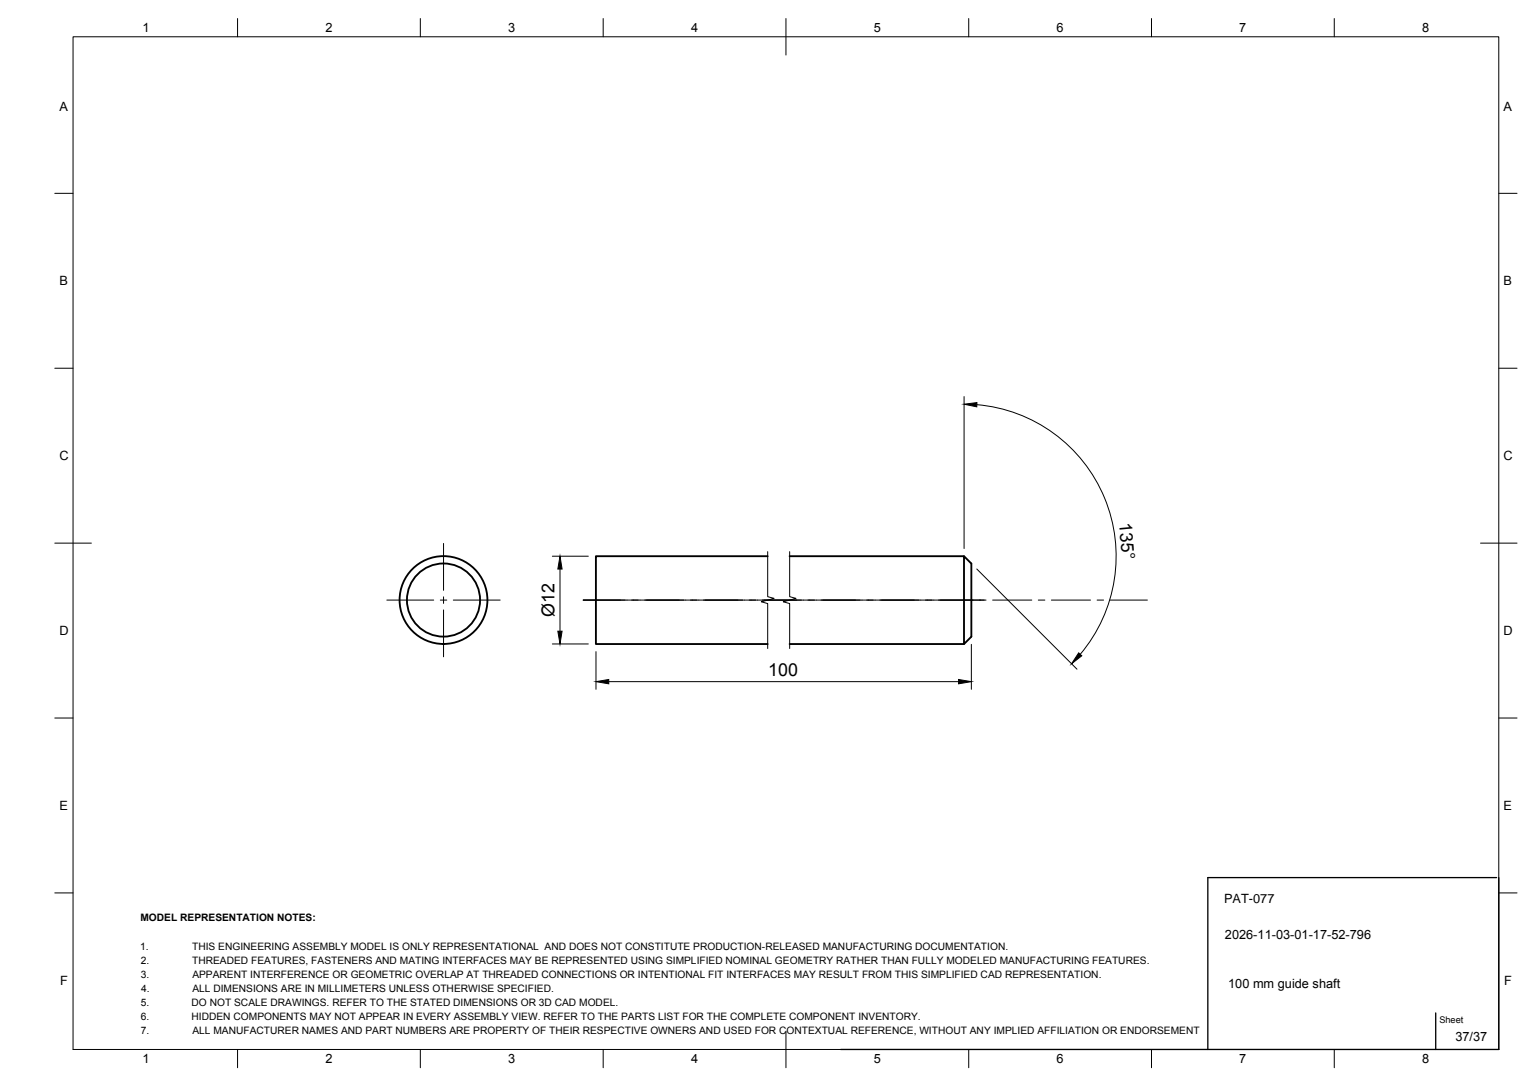
ISO-10303-21;
HEADER;
/* Generated by software containing ST-Developer
 * from STEP Tools, Inc. (www.steptools.com) 
 */

FILE_DESCRIPTION(
/* description */ ('Pallet stop with pneumatic fitting'),
/* implementation_level */ '2;1');

FILE_NAME(
/* name */ '100 mm guide shaft.step',
/* time_stamp */ '2026-10-27T10:51:41-07:00',
/* author */ (''),
/* organization */ (''),
/* preprocessor_version */ 'ST-DEVELOPER v20.2',
/* originating_system */ 'Autodesk Translation Framework v15.17.0.0',
/* authorisation */ '');

FILE_SCHEMA (('AUTOMOTIVE_DESIGN { 1 0 10303 214 3 1 1 }'));
ENDSEC;

DATA;
#10=MECHANICAL_DESIGN_GEOMETRIC_PRESENTATION_REPRESENTATION('',(#386),#10265);
#32=CONICAL_SURFACE('',#5987,0.55,0.785398163397448);
#322=SHAPE_REPRESENTATION_RELATIONSHIP('SRR','None',#10438,#354);
#354=ADVANCED_BREP_SHAPE_REPRESENTATION('',(#417),#10262);
#386=STYLED_ITEM('',(#10655),#417);
#417=MANIFOLD_SOLID_BREP('Body1',#5075);
#714=PLANE('',#5985);
#715=PLANE('',#5991);
#1018=FACE_OUTER_BOUND('',#1456,.T.);
#1019=FACE_OUTER_BOUND('',#1457,.T.);
#1020=FACE_OUTER_BOUND('',#1458,.T.);
#1021=FACE_OUTER_BOUND('',#1459,.T.);
#1456=EDGE_LOOP('',(#4502));
#1457=EDGE_LOOP('',(#4503,#4504,#4505,#4506));
#1458=EDGE_LOOP('',(#4507,#4508,#4509,#4510));
#1459=EDGE_LOOP('',(#4511));
#1779=LINE('',#10009,#2114);
#1780=LINE('',#10012,#2115);
#2114=VECTOR('',#7492,0.55);
#2115=VECTOR('',#7497,0.6);
#2393=CIRCLE('',#5986,0.6);
#2394=CIRCLE('',#5988,0.6);
#2395=CIRCLE('',#5989,0.5);
#2766=VERTEX_POINT('',#10003);
#2767=VERTEX_POINT('',#10006);
#2768=VERTEX_POINT('',#10008);
#3350=EDGE_CURVE('',#2766,#2766,#2393,.T.);
#3351=EDGE_CURVE('',#2767,#2767,#2394,.T.);
#3352=EDGE_CURVE('',#2767,#2768,#1779,.T.);
#3353=EDGE_CURVE('',#2768,#2768,#2395,.T.);
#3354=EDGE_CURVE('',#2766,#2767,#1780,.T.);
#4502=ORIENTED_EDGE('',*,*,#3350,.F.);
#4503=ORIENTED_EDGE('',*,*,#3351,.T.);
#4504=ORIENTED_EDGE('',*,*,#3352,.T.);
#4505=ORIENTED_EDGE('',*,*,#3353,.T.);
#4506=ORIENTED_EDGE('',*,*,#3352,.F.);
#4507=ORIENTED_EDGE('',*,*,#3350,.T.);
#4508=ORIENTED_EDGE('',*,*,#3354,.T.);
#4509=ORIENTED_EDGE('',*,*,#3351,.F.);
#4510=ORIENTED_EDGE('',*,*,#3354,.F.);
#4511=ORIENTED_EDGE('',*,*,#3353,.F.);
#4727=CYLINDRICAL_SURFACE('',#5990,0.6);
#5013=ADVANCED_FACE('',(#1018),#714,.T.);
#5014=ADVANCED_FACE('',(#1019),#32,.T.);
#5015=ADVANCED_FACE('',(#1020),#4727,.T.);
#5016=ADVANCED_FACE('',(#1021),#715,.F.);
#5075=CLOSED_SHELL('',(#5013,#5014,#5015,#5016));
#5984=AXIS2_PLACEMENT_3D('',#10001,#7482,#7483);
#5985=AXIS2_PLACEMENT_3D('',#10002,#7484,#7485);
#5986=AXIS2_PLACEMENT_3D('',#10004,#7486,#7487);
#5987=AXIS2_PLACEMENT_3D('',#10005,#7488,#7489);
#5988=AXIS2_PLACEMENT_3D('',#10007,#7490,#7491);
#5989=AXIS2_PLACEMENT_3D('',#10010,#7493,#7494);
#5990=AXIS2_PLACEMENT_3D('',#10011,#7495,#7496);
#5991=AXIS2_PLACEMENT_3D('',#10013,#7498,#7499);
#7482=DIRECTION('axis',(0.,0.,1.));
#7483=DIRECTION('refdir',(1.,0.,0.));
#7484=DIRECTION('center_axis',(1.,0.,0.));
#7485=DIRECTION('ref_axis',(0.,0.,-1.));
#7486=DIRECTION('center_axis',(-1.,0.,0.));
#7487=DIRECTION('ref_axis',(0.,0.,-1.));
#7488=DIRECTION('center_axis',(1.,0.,0.));
#7489=DIRECTION('ref_axis',(0.,0.,-1.));
#7490=DIRECTION('center_axis',(-1.,0.,0.));
#7491=DIRECTION('ref_axis',(0.,0.,-1.));
#7492=DIRECTION('',(-0.707106781186548,8.65956056235493E-17,-0.707106781186547));
#7493=DIRECTION('center_axis',(1.,0.,0.));
#7494=DIRECTION('ref_axis',(0.,0.,-1.));
#7495=DIRECTION('center_axis',(1.,0.,0.));
#7496=DIRECTION('ref_axis',(0.,0.,-1.));
#7497=DIRECTION('',(-1.,0.,0.));
#7498=DIRECTION('center_axis',(1.,0.,0.));
#7499=DIRECTION('ref_axis',(0.,0.,-1.));
#10001=CARTESIAN_POINT('',(0.,0.,0.));
#10002=CARTESIAN_POINT('Origin',(10.,0.,0.));
#10003=CARTESIAN_POINT('',(10.,7.34788079488412E-17,0.6));
#10004=CARTESIAN_POINT('Origin',(10.,0.,0.));
#10005=CARTESIAN_POINT('Origin',(0.05,0.,0.));
#10006=CARTESIAN_POINT('',(0.1,7.34788079488412E-17,0.6));
#10007=CARTESIAN_POINT('Origin',(0.1,0.,0.));
#10008=CARTESIAN_POINT('',(0.,-6.12323399573677E-17,0.5));
#10009=CARTESIAN_POINT('',(0.05,-6.73555739531044E-17,0.55));
#10010=CARTESIAN_POINT('Origin',(0.,0.,0.));
#10011=CARTESIAN_POINT('Origin',(0.,0.,0.));
#10012=CARTESIAN_POINT('',(0.,-7.34788079488412E-17,0.6));
#10013=CARTESIAN_POINT('Origin',(0.,0.,0.));
#10224=UNCERTAINTY_MEASURE_WITH_UNIT(LENGTH_MEASURE(0.001),#10266,
'DISTANCE_ACCURACY_VALUE',
'Maximum model space distance between geometric entities at asserted c
onnectivities');
#10227=UNCERTAINTY_MEASURE_WITH_UNIT(LENGTH_MEASURE(0.001),#10266,
'DISTANCE_ACCURACY_VALUE',
'Maximum model space distance between geometric entities at asserted c
onnectivities');
#10262=(
GEOMETRIC_REPRESENTATION_CONTEXT(3)
GLOBAL_UNCERTAINTY_ASSIGNED_CONTEXT((#10224))
GLOBAL_UNIT_ASSIGNED_CONTEXT((#10266,#10268,#10269))
REPRESENTATION_CONTEXT('','3D')
);
#10265=(
GEOMETRIC_REPRESENTATION_CONTEXT(3)
GLOBAL_UNCERTAINTY_ASSIGNED_CONTEXT((#10227))
GLOBAL_UNIT_ASSIGNED_CONTEXT((#10266,#10268,#10269))
REPRESENTATION_CONTEXT('','3D')
);
#10266=(
LENGTH_UNIT()
NAMED_UNIT(*)
SI_UNIT(.CENTI.,.METRE.)
);
#10268=(
NAMED_UNIT(*)
PLANE_ANGLE_UNIT()
SI_UNIT($,.RADIAN.)
);
#10269=(
NAMED_UNIT(*)
SI_UNIT($,.STERADIAN.)
SOLID_ANGLE_UNIT()
);
#10304=SHAPE_DEFINITION_REPRESENTATION(#10345,#10438);
#10345=PRODUCT_DEFINITION_SHAPE('',$,#10476);
#10438=SHAPE_REPRESENTATION('',(#5984),#10262);
#10441=PRODUCT_DEFINITION_CONTEXT('part definition',#10554,'design');
#10476=PRODUCT_DEFINITION('100 mm guide shaft','100 mm guide shaft',#10513,
#10441);
#10513=PRODUCT_DEFINITION_FORMATION('',$,#10590);
#10554=APPLICATION_CONTEXT(
'Core Data for Automotive Mechanical Design Process');
#10555=PRODUCT_CONTEXT('part definition',#10554,'mechanical');
#10590=PRODUCT('100 mm guide shaft','100 mm guide shaft',
'100 mm guide shaft',(#10555));
#10649=COLOUR_RGB('Grey',0.48,0.52,0.57);
#10650=FILL_AREA_STYLE_COLOUR('',#10649);
#10651=FILL_AREA_STYLE('',(#10650));
#10652=SURFACE_STYLE_FILL_AREA(#10651);
#10653=SURFACE_SIDE_STYLE('',(#10652));
#10654=SURFACE_STYLE_USAGE(.BOTH.,#10653);
#10655=PRESENTATION_STYLE_ASSIGNMENT((#10654));
ENDSEC;
END-ISO-10303-21;
